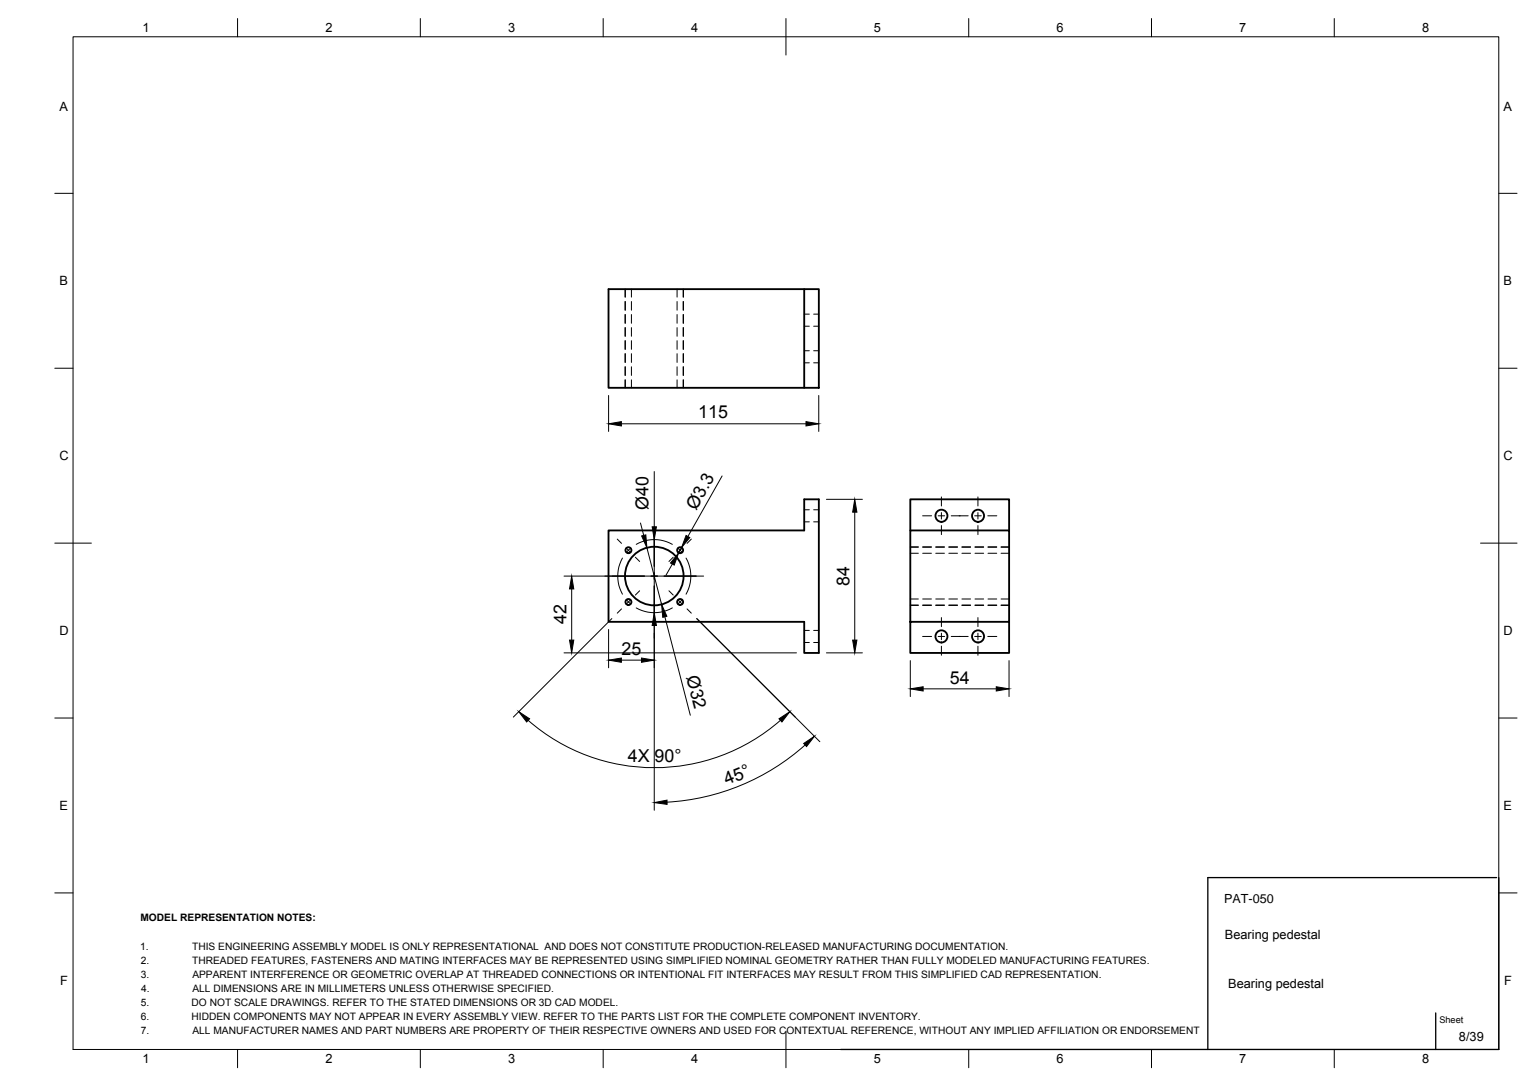
ISO-10303-21;
HEADER;
/* Generated by software containing ST-Developer
 * from STEP Tools, Inc. (www.steptools.com) 
 */

FILE_DESCRIPTION(
/* description */ ('Hand wheel with handle and shaft collar'),
/* implementation_level */ '2;1');

FILE_NAME(
/* name */ 'Bearing pedestal.step',
/* time_stamp */ '2026-10-28T03:23:19-07:00',
/* author */ (''),
/* organization */ (''),
/* preprocessor_version */ 'ST-DEVELOPER v20.2',
/* originating_system */ 'Autodesk Translation Framework v15.17.0.0',
/* authorisation */ '');

FILE_SCHEMA (('AUTOMOTIVE_DESIGN { 1 0 10303 214 3 1 1 }'));
ENDSEC;

DATA;
#10=MECHANICAL_DESIGN_GEOMETRIC_PRESENTATION_REPRESENTATION('',(#398),#10510);
#334=SHAPE_REPRESENTATION_RELATIONSHIP('SRR','None',#10650,#366);
#366=ADVANCED_BREP_SHAPE_REPRESENTATION('',(#445),#10477);
#398=STYLED_ITEM('',(#10908),#445);
#445=MANIFOLD_SOLID_BREP('Body1',#5297);
#494=FACE_BOUND('',#1122,.T.);
#495=FACE_BOUND('',#1123,.T.);
#496=FACE_BOUND('',#1125,.T.);
#497=FACE_BOUND('',#1126,.T.);
#498=FACE_BOUND('',#1130,.T.);
#499=FACE_BOUND('',#1131,.T.);
#500=FACE_BOUND('',#1132,.T.);
#501=FACE_BOUND('',#1133,.T.);
#502=FACE_BOUND('',#1134,.T.);
#503=FACE_BOUND('',#1137,.T.);
#504=FACE_BOUND('',#1138,.T.);
#505=FACE_BOUND('',#1139,.T.);
#506=FACE_BOUND('',#1140,.T.);
#507=FACE_BOUND('',#1141,.T.);
#508=FACE_BOUND('',#1145,.T.);
#509=FACE_BOUND('',#1146,.T.);
#510=FACE_BOUND('',#1147,.T.);
#511=FACE_BOUND('',#1148,.T.);
#616=PLANE('',#5760);
#617=PLANE('',#5761);
#618=PLANE('',#5762);
#619=PLANE('',#5763);
#620=PLANE('',#5764);
#621=PLANE('',#5765);
#622=PLANE('',#5766);
#623=PLANE('',#5767);
#624=PLANE('',#5768);
#625=PLANE('',#5769);
#785=FACE_OUTER_BOUND('',#1112,.T.);
#786=FACE_OUTER_BOUND('',#1113,.T.);
#787=FACE_OUTER_BOUND('',#1114,.T.);
#788=FACE_OUTER_BOUND('',#1115,.T.);
#789=FACE_OUTER_BOUND('',#1116,.T.);
#790=FACE_OUTER_BOUND('',#1117,.T.);
#791=FACE_OUTER_BOUND('',#1118,.T.);
#792=FACE_OUTER_BOUND('',#1119,.T.);
#793=FACE_OUTER_BOUND('',#1120,.T.);
#794=FACE_OUTER_BOUND('',#1121,.T.);
#795=FACE_OUTER_BOUND('',#1124,.T.);
#796=FACE_OUTER_BOUND('',#1127,.T.);
#797=FACE_OUTER_BOUND('',#1128,.T.);
#798=FACE_OUTER_BOUND('',#1129,.T.);
#799=FACE_OUTER_BOUND('',#1135,.T.);
#800=FACE_OUTER_BOUND('',#1136,.T.);
#801=FACE_OUTER_BOUND('',#1142,.T.);
#802=FACE_OUTER_BOUND('',#1143,.T.);
#803=FACE_OUTER_BOUND('',#1144,.T.);
#1112=EDGE_LOOP('',(#3653,#3654,#3655,#3656));
#1113=EDGE_LOOP('',(#3657,#3658,#3659,#3660));
#1114=EDGE_LOOP('',(#3661,#3662,#3663,#3664));
#1115=EDGE_LOOP('',(#3665,#3666,#3667,#3668));
#1116=EDGE_LOOP('',(#3669,#3670,#3671,#3672));
#1117=EDGE_LOOP('',(#3673,#3674,#3675,#3676));
#1118=EDGE_LOOP('',(#3677,#3678,#3679,#3680));
#1119=EDGE_LOOP('',(#3681,#3682,#3683,#3684));
#1120=EDGE_LOOP('',(#3685,#3686,#3687,#3688));
#1121=EDGE_LOOP('',(#3689,#3690,#3691,#3692));
#1122=EDGE_LOOP('',(#3693));
#1123=EDGE_LOOP('',(#3694));
#1124=EDGE_LOOP('',(#3695,#3696,#3697,#3698));
#1125=EDGE_LOOP('',(#3699));
#1126=EDGE_LOOP('',(#3700));
#1127=EDGE_LOOP('',(#3701,#3702,#3703,#3704));
#1128=EDGE_LOOP('',(#3705,#3706,#3707,#3708));
#1129=EDGE_LOOP('',(#3709,#3710,#3711,#3712,#3713,#3714,#3715,#3716));
#1130=EDGE_LOOP('',(#3717));
#1131=EDGE_LOOP('',(#3718));
#1132=EDGE_LOOP('',(#3719));
#1133=EDGE_LOOP('',(#3720));
#1134=EDGE_LOOP('',(#3721));
#1135=EDGE_LOOP('',(#3722,#3723,#3724,#3725));
#1136=EDGE_LOOP('',(#3726,#3727,#3728,#3729,#3730,#3731,#3732,#3733));
#1137=EDGE_LOOP('',(#3734));
#1138=EDGE_LOOP('',(#3735));
#1139=EDGE_LOOP('',(#3736));
#1140=EDGE_LOOP('',(#3737));
#1141=EDGE_LOOP('',(#3738));
#1142=EDGE_LOOP('',(#3739,#3740,#3741,#3742));
#1143=EDGE_LOOP('',(#3743,#3744,#3745,#3746));
#1144=EDGE_LOOP('',(#3747,#3748,#3749,#3750));
#1145=EDGE_LOOP('',(#3751));
#1146=EDGE_LOOP('',(#3752));
#1147=EDGE_LOOP('',(#3753));
#1148=EDGE_LOOP('',(#3754));
#1553=LINE('',#8285,#1863);
#1554=LINE('',#8291,#1864);
#1555=LINE('',#8297,#1865);
#1556=LINE('',#8303,#1866);
#1557=LINE('',#8309,#1867);
#1558=LINE('',#8315,#1868);
#1559=LINE('',#8321,#1869);
#1560=LINE('',#8327,#1870);
#1561=LINE('',#8333,#1871);
#1562=LINE('',#8338,#1872);
#1563=LINE('',#8340,#1873);
#1564=LINE('',#8342,#1874);
#1565=LINE('',#8343,#1875);
#1566=LINE('',#8347,#1876);
#1567=LINE('',#8349,#1877);
#1568=LINE('',#8351,#1878);
#1569=LINE('',#8352,#1879);
#1570=LINE('',#8355,#1880);
#1571=LINE('',#8357,#1881);
#1572=LINE('',#8358,#1882);
#1573=LINE('',#8361,#1883);
#1574=LINE('',#8363,#1884);
#1575=LINE('',#8364,#1885);
#1576=LINE('',#8367,#1886);
#1577=LINE('',#8369,#1887);
#1578=LINE('',#8370,#1888);
#1579=LINE('',#8371,#1889);
#1580=LINE('',#8374,#1890);
#1581=LINE('',#8375,#1891);
#1582=LINE('',#8378,#1892);
#1583=LINE('',#8379,#1893);
#1584=LINE('',#8380,#1894);
#1585=LINE('',#8382,#1895);
#1863=VECTOR('',#6535,0.165);
#1864=VECTOR('',#6542,0.165);
#1865=VECTOR('',#6549,0.165);
#1866=VECTOR('',#6556,0.165);
#1867=VECTOR('',#6563,0.33);
#1868=VECTOR('',#6570,0.33);
#1869=VECTOR('',#6577,0.33);
#1870=VECTOR('',#6584,0.33);
#1871=VECTOR('',#6591,1.6);
#1872=VECTOR('',#6596,1.);
#1873=VECTOR('',#6597,1.);
#1874=VECTOR('',#6598,1.);
#1875=VECTOR('',#6599,1.);
#1876=VECTOR('',#6602,1.);
#1877=VECTOR('',#6603,1.);
#1878=VECTOR('',#6604,1.);
#1879=VECTOR('',#6605,1.);
#1880=VECTOR('',#6608,1.);
#1881=VECTOR('',#6609,1.);
#1882=VECTOR('',#6610,1.);
#1883=VECTOR('',#6613,1.);
#1884=VECTOR('',#6614,1.);
#1885=VECTOR('',#6615,1.);
#1886=VECTOR('',#6618,1.);
#1887=VECTOR('',#6619,1.);
#1888=VECTOR('',#6620,1.);
#1889=VECTOR('',#6621,1.);
#1890=VECTOR('',#6624,1.);
#1891=VECTOR('',#6625,1.);
#1892=VECTOR('',#6628,1.);
#1893=VECTOR('',#6629,1.);
#1894=VECTOR('',#6630,1.);
#1895=VECTOR('',#6633,1.);
#2141=CIRCLE('',#5734,0.165);
#2142=CIRCLE('',#5735,0.165);
#2143=CIRCLE('',#5737,0.165);
#2144=CIRCLE('',#5738,0.165);
#2145=CIRCLE('',#5740,0.165);
#2146=CIRCLE('',#5741,0.165);
#2147=CIRCLE('',#5743,0.165);
#2148=CIRCLE('',#5744,0.165);
#2149=CIRCLE('',#5746,0.33);
#2150=CIRCLE('',#5747,0.33);
#2151=CIRCLE('',#5749,0.33);
#2152=CIRCLE('',#5750,0.33);
#2153=CIRCLE('',#5752,0.33);
#2154=CIRCLE('',#5753,0.33);
#2155=CIRCLE('',#5755,0.33);
#2156=CIRCLE('',#5756,0.33);
#2157=CIRCLE('',#5758,1.6);
#2158=CIRCLE('',#5759,1.6);
#2476=VERTEX_POINT('',#8282);
#2477=VERTEX_POINT('',#8284);
#2478=VERTEX_POINT('',#8288);
#2479=VERTEX_POINT('',#8290);
#2480=VERTEX_POINT('',#8294);
#2481=VERTEX_POINT('',#8296);
#2482=VERTEX_POINT('',#8300);
#2483=VERTEX_POINT('',#8302);
#2484=VERTEX_POINT('',#8306);
#2485=VERTEX_POINT('',#8308);
#2486=VERTEX_POINT('',#8312);
#2487=VERTEX_POINT('',#8314);
#2488=VERTEX_POINT('',#8318);
#2489=VERTEX_POINT('',#8320);
#2490=VERTEX_POINT('',#8324);
#2491=VERTEX_POINT('',#8326);
#2492=VERTEX_POINT('',#8330);
#2493=VERTEX_POINT('',#8332);
#2494=VERTEX_POINT('',#8336);
#2495=VERTEX_POINT('',#8337);
#2496=VERTEX_POINT('',#8339);
#2497=VERTEX_POINT('',#8341);
#2498=VERTEX_POINT('',#8345);
#2499=VERTEX_POINT('',#8346);
#2500=VERTEX_POINT('',#8348);
#2501=VERTEX_POINT('',#8350);
#2502=VERTEX_POINT('',#8354);
#2503=VERTEX_POINT('',#8356);
#2504=VERTEX_POINT('',#8360);
#2505=VERTEX_POINT('',#8362);
#2506=VERTEX_POINT('',#8366);
#2507=VERTEX_POINT('',#8368);
#2508=VERTEX_POINT('',#8373);
#2509=VERTEX_POINT('',#8377);
#2944=EDGE_CURVE('',#2476,#2476,#2141,.T.);
#2945=EDGE_CURVE('',#2476,#2477,#1553,.T.);
#2946=EDGE_CURVE('',#2477,#2477,#2142,.T.);
#2947=EDGE_CURVE('',#2478,#2478,#2143,.T.);
#2948=EDGE_CURVE('',#2478,#2479,#1554,.T.);
#2949=EDGE_CURVE('',#2479,#2479,#2144,.T.);
#2950=EDGE_CURVE('',#2480,#2480,#2145,.T.);
#2951=EDGE_CURVE('',#2480,#2481,#1555,.T.);
#2952=EDGE_CURVE('',#2481,#2481,#2146,.T.);
#2953=EDGE_CURVE('',#2482,#2482,#2147,.T.);
#2954=EDGE_CURVE('',#2482,#2483,#1556,.T.);
#2955=EDGE_CURVE('',#2483,#2483,#2148,.T.);
#2956=EDGE_CURVE('',#2484,#2484,#2149,.T.);
#2957=EDGE_CURVE('',#2484,#2485,#1557,.T.);
#2958=EDGE_CURVE('',#2485,#2485,#2150,.T.);
#2959=EDGE_CURVE('',#2486,#2486,#2151,.T.);
#2960=EDGE_CURVE('',#2486,#2487,#1558,.T.);
#2961=EDGE_CURVE('',#2487,#2487,#2152,.T.);
#2962=EDGE_CURVE('',#2488,#2488,#2153,.T.);
#2963=EDGE_CURVE('',#2488,#2489,#1559,.T.);
#2964=EDGE_CURVE('',#2489,#2489,#2154,.T.);
#2965=EDGE_CURVE('',#2490,#2490,#2155,.T.);
#2966=EDGE_CURVE('',#2490,#2491,#1560,.T.);
#2967=EDGE_CURVE('',#2491,#2491,#2156,.T.);
#2968=EDGE_CURVE('',#2492,#2492,#2157,.T.);
#2969=EDGE_CURVE('',#2492,#2493,#1561,.T.);
#2970=EDGE_CURVE('',#2493,#2493,#2158,.T.);
#2971=EDGE_CURVE('',#2494,#2495,#1562,.T.);
#2972=EDGE_CURVE('',#2496,#2494,#1563,.T.);
#2973=EDGE_CURVE('',#2496,#2497,#1564,.T.);
#2974=EDGE_CURVE('',#2495,#2497,#1565,.T.);
#2975=EDGE_CURVE('',#2498,#2499,#1566,.T.);
#2976=EDGE_CURVE('',#2500,#2498,#1567,.T.);
#2977=EDGE_CURVE('',#2501,#2500,#1568,.T.);
#2978=EDGE_CURVE('',#2499,#2501,#1569,.T.);
#2979=EDGE_CURVE('',#2501,#2502,#1570,.T.);
#2980=EDGE_CURVE('',#2503,#2500,#1571,.T.);
#2981=EDGE_CURVE('',#2502,#2503,#1572,.T.);
#2982=EDGE_CURVE('',#2504,#2496,#1573,.T.);
#2983=EDGE_CURVE('',#2504,#2505,#1574,.T.);
#2984=EDGE_CURVE('',#2497,#2505,#1575,.T.);
#2985=EDGE_CURVE('',#2494,#2506,#1576,.T.);
#2986=EDGE_CURVE('',#2507,#2506,#1577,.T.);
#2987=EDGE_CURVE('',#2499,#2507,#1578,.T.);
#2988=EDGE_CURVE('',#2502,#2504,#1579,.T.);
#2989=EDGE_CURVE('',#2495,#2508,#1580,.T.);
#2990=EDGE_CURVE('',#2506,#2508,#1581,.T.);
#2991=EDGE_CURVE('',#2498,#2509,#1582,.T.);
#2992=EDGE_CURVE('',#2508,#2509,#1583,.T.);
#2993=EDGE_CURVE('',#2505,#2503,#1584,.T.);
#2994=EDGE_CURVE('',#2509,#2507,#1585,.T.);
#3653=ORIENTED_EDGE('',*,*,#2944,.F.);
#3654=ORIENTED_EDGE('',*,*,#2945,.T.);
#3655=ORIENTED_EDGE('',*,*,#2946,.F.);
#3656=ORIENTED_EDGE('',*,*,#2945,.F.);
#3657=ORIENTED_EDGE('',*,*,#2947,.F.);
#3658=ORIENTED_EDGE('',*,*,#2948,.T.);
#3659=ORIENTED_EDGE('',*,*,#2949,.F.);
#3660=ORIENTED_EDGE('',*,*,#2948,.F.);
#3661=ORIENTED_EDGE('',*,*,#2950,.F.);
#3662=ORIENTED_EDGE('',*,*,#2951,.T.);
#3663=ORIENTED_EDGE('',*,*,#2952,.F.);
#3664=ORIENTED_EDGE('',*,*,#2951,.F.);
#3665=ORIENTED_EDGE('',*,*,#2953,.F.);
#3666=ORIENTED_EDGE('',*,*,#2954,.T.);
#3667=ORIENTED_EDGE('',*,*,#2955,.F.);
#3668=ORIENTED_EDGE('',*,*,#2954,.F.);
#3669=ORIENTED_EDGE('',*,*,#2956,.F.);
#3670=ORIENTED_EDGE('',*,*,#2957,.T.);
#3671=ORIENTED_EDGE('',*,*,#2958,.F.);
#3672=ORIENTED_EDGE('',*,*,#2957,.F.);
#3673=ORIENTED_EDGE('',*,*,#2959,.F.);
#3674=ORIENTED_EDGE('',*,*,#2960,.T.);
#3675=ORIENTED_EDGE('',*,*,#2961,.F.);
#3676=ORIENTED_EDGE('',*,*,#2960,.F.);
#3677=ORIENTED_EDGE('',*,*,#2962,.F.);
#3678=ORIENTED_EDGE('',*,*,#2963,.T.);
#3679=ORIENTED_EDGE('',*,*,#2964,.F.);
#3680=ORIENTED_EDGE('',*,*,#2963,.F.);
#3681=ORIENTED_EDGE('',*,*,#2965,.F.);
#3682=ORIENTED_EDGE('',*,*,#2966,.T.);
#3683=ORIENTED_EDGE('',*,*,#2967,.F.);
#3684=ORIENTED_EDGE('',*,*,#2966,.F.);
#3685=ORIENTED_EDGE('',*,*,#2968,.F.);
#3686=ORIENTED_EDGE('',*,*,#2969,.T.);
#3687=ORIENTED_EDGE('',*,*,#2970,.F.);
#3688=ORIENTED_EDGE('',*,*,#2969,.F.);
#3689=ORIENTED_EDGE('',*,*,#2971,.F.);
#3690=ORIENTED_EDGE('',*,*,#2972,.F.);
#3691=ORIENTED_EDGE('',*,*,#2973,.T.);
#3692=ORIENTED_EDGE('',*,*,#2974,.F.);
#3693=ORIENTED_EDGE('',*,*,#2958,.T.);
#3694=ORIENTED_EDGE('',*,*,#2967,.T.);
#3695=ORIENTED_EDGE('',*,*,#2975,.F.);
#3696=ORIENTED_EDGE('',*,*,#2976,.F.);
#3697=ORIENTED_EDGE('',*,*,#2977,.F.);
#3698=ORIENTED_EDGE('',*,*,#2978,.F.);
#3699=ORIENTED_EDGE('',*,*,#2961,.T.);
#3700=ORIENTED_EDGE('',*,*,#2964,.T.);
#3701=ORIENTED_EDGE('',*,*,#2979,.F.);
#3702=ORIENTED_EDGE('',*,*,#2977,.T.);
#3703=ORIENTED_EDGE('',*,*,#2980,.F.);
#3704=ORIENTED_EDGE('',*,*,#2981,.F.);
#3705=ORIENTED_EDGE('',*,*,#2982,.F.);
#3706=ORIENTED_EDGE('',*,*,#2983,.T.);
#3707=ORIENTED_EDGE('',*,*,#2984,.F.);
#3708=ORIENTED_EDGE('',*,*,#2973,.F.);
#3709=ORIENTED_EDGE('',*,*,#2985,.T.);
#3710=ORIENTED_EDGE('',*,*,#2986,.F.);
#3711=ORIENTED_EDGE('',*,*,#2987,.F.);
#3712=ORIENTED_EDGE('',*,*,#2978,.T.);
#3713=ORIENTED_EDGE('',*,*,#2979,.T.);
#3714=ORIENTED_EDGE('',*,*,#2988,.T.);
#3715=ORIENTED_EDGE('',*,*,#2982,.T.);
#3716=ORIENTED_EDGE('',*,*,#2972,.T.);
#3717=ORIENTED_EDGE('',*,*,#2968,.T.);
#3718=ORIENTED_EDGE('',*,*,#2953,.T.);
#3719=ORIENTED_EDGE('',*,*,#2950,.T.);
#3720=ORIENTED_EDGE('',*,*,#2947,.T.);
#3721=ORIENTED_EDGE('',*,*,#2944,.T.);
#3722=ORIENTED_EDGE('',*,*,#2971,.T.);
#3723=ORIENTED_EDGE('',*,*,#2989,.T.);
#3724=ORIENTED_EDGE('',*,*,#2990,.F.);
#3725=ORIENTED_EDGE('',*,*,#2985,.F.);
#3726=ORIENTED_EDGE('',*,*,#2991,.T.);
#3727=ORIENTED_EDGE('',*,*,#2992,.F.);
#3728=ORIENTED_EDGE('',*,*,#2989,.F.);
#3729=ORIENTED_EDGE('',*,*,#2974,.T.);
#3730=ORIENTED_EDGE('',*,*,#2984,.T.);
#3731=ORIENTED_EDGE('',*,*,#2993,.T.);
#3732=ORIENTED_EDGE('',*,*,#2980,.T.);
#3733=ORIENTED_EDGE('',*,*,#2976,.T.);
#3734=ORIENTED_EDGE('',*,*,#2970,.T.);
#3735=ORIENTED_EDGE('',*,*,#2955,.T.);
#3736=ORIENTED_EDGE('',*,*,#2952,.T.);
#3737=ORIENTED_EDGE('',*,*,#2949,.T.);
#3738=ORIENTED_EDGE('',*,*,#2946,.T.);
#3739=ORIENTED_EDGE('',*,*,#2975,.T.);
#3740=ORIENTED_EDGE('',*,*,#2987,.T.);
#3741=ORIENTED_EDGE('',*,*,#2994,.F.);
#3742=ORIENTED_EDGE('',*,*,#2991,.F.);
#3743=ORIENTED_EDGE('',*,*,#2994,.T.);
#3744=ORIENTED_EDGE('',*,*,#2986,.T.);
#3745=ORIENTED_EDGE('',*,*,#2990,.T.);
#3746=ORIENTED_EDGE('',*,*,#2992,.T.);
#3747=ORIENTED_EDGE('',*,*,#2993,.F.);
#3748=ORIENTED_EDGE('',*,*,#2983,.F.);
#3749=ORIENTED_EDGE('',*,*,#2988,.F.);
#3750=ORIENTED_EDGE('',*,*,#2981,.T.);
#3751=ORIENTED_EDGE('',*,*,#2956,.T.);
#3752=ORIENTED_EDGE('',*,*,#2959,.T.);
#3753=ORIENTED_EDGE('',*,*,#2962,.T.);
#3754=ORIENTED_EDGE('',*,*,#2965,.T.);
#4883=CYLINDRICAL_SURFACE('',#5733,0.165);
#4884=CYLINDRICAL_SURFACE('',#5736,0.165);
#4885=CYLINDRICAL_SURFACE('',#5739,0.165);
#4886=CYLINDRICAL_SURFACE('',#5742,0.165);
#4887=CYLINDRICAL_SURFACE('',#5745,0.33);
#4888=CYLINDRICAL_SURFACE('',#5748,0.33);
#4889=CYLINDRICAL_SURFACE('',#5751,0.33);
#4890=CYLINDRICAL_SURFACE('',#5754,0.33);
#4891=CYLINDRICAL_SURFACE('',#5757,1.6);
#4997=ADVANCED_FACE('',(#785),#4883,.F.);
#4998=ADVANCED_FACE('',(#786),#4884,.F.);
#4999=ADVANCED_FACE('',(#787),#4885,.F.);
#5000=ADVANCED_FACE('',(#788),#4886,.F.);
#5001=ADVANCED_FACE('',(#789),#4887,.F.);
#5002=ADVANCED_FACE('',(#790),#4888,.F.);
#5003=ADVANCED_FACE('',(#791),#4889,.F.);
#5004=ADVANCED_FACE('',(#792),#4890,.F.);
#5005=ADVANCED_FACE('',(#793),#4891,.F.);
#5006=ADVANCED_FACE('',(#794,#494,#495),#616,.T.);
#5007=ADVANCED_FACE('',(#795,#496,#497),#617,.T.);
#5008=ADVANCED_FACE('',(#796),#618,.T.);
#5009=ADVANCED_FACE('',(#797),#619,.T.);
#5010=ADVANCED_FACE('',(#798,#498,#499,#500,#501,#502),#620,.T.);
#5011=ADVANCED_FACE('',(#799),#621,.T.);
#5012=ADVANCED_FACE('',(#800,#503,#504,#505,#506,#507),#622,.T.);
#5013=ADVANCED_FACE('',(#801),#623,.T.);
#5014=ADVANCED_FACE('',(#802),#624,.T.);
#5015=ADVANCED_FACE('',(#803,#508,#509,#510,#511),#625,.F.);
#5297=CLOSED_SHELL('',(#4997,#4998,#4999,#5000,#5001,#5002,#5003,#5004,
#5005,#5006,#5007,#5008,#5009,#5010,#5011,#5012,#5013,#5014,#5015));
#5732=AXIS2_PLACEMENT_3D('',#8280,#6529,#6530);
#5733=AXIS2_PLACEMENT_3D('',#8281,#6531,#6532);
#5734=AXIS2_PLACEMENT_3D('',#8283,#6533,#6534);
#5735=AXIS2_PLACEMENT_3D('',#8286,#6536,#6537);
#5736=AXIS2_PLACEMENT_3D('',#8287,#6538,#6539);
#5737=AXIS2_PLACEMENT_3D('',#8289,#6540,#6541);
#5738=AXIS2_PLACEMENT_3D('',#8292,#6543,#6544);
#5739=AXIS2_PLACEMENT_3D('',#8293,#6545,#6546);
#5740=AXIS2_PLACEMENT_3D('',#8295,#6547,#6548);
#5741=AXIS2_PLACEMENT_3D('',#8298,#6550,#6551);
#5742=AXIS2_PLACEMENT_3D('',#8299,#6552,#6553);
#5743=AXIS2_PLACEMENT_3D('',#8301,#6554,#6555);
#5744=AXIS2_PLACEMENT_3D('',#8304,#6557,#6558);
#5745=AXIS2_PLACEMENT_3D('',#8305,#6559,#6560);
#5746=AXIS2_PLACEMENT_3D('',#8307,#6561,#6562);
#5747=AXIS2_PLACEMENT_3D('',#8310,#6564,#6565);
#5748=AXIS2_PLACEMENT_3D('',#8311,#6566,#6567);
#5749=AXIS2_PLACEMENT_3D('',#8313,#6568,#6569);
#5750=AXIS2_PLACEMENT_3D('',#8316,#6571,#6572);
#5751=AXIS2_PLACEMENT_3D('',#8317,#6573,#6574);
#5752=AXIS2_PLACEMENT_3D('',#8319,#6575,#6576);
#5753=AXIS2_PLACEMENT_3D('',#8322,#6578,#6579);
#5754=AXIS2_PLACEMENT_3D('',#8323,#6580,#6581);
#5755=AXIS2_PLACEMENT_3D('',#8325,#6582,#6583);
#5756=AXIS2_PLACEMENT_3D('',#8328,#6585,#6586);
#5757=AXIS2_PLACEMENT_3D('',#8329,#6587,#6588);
#5758=AXIS2_PLACEMENT_3D('',#8331,#6589,#6590);
#5759=AXIS2_PLACEMENT_3D('',#8334,#6592,#6593);
#5760=AXIS2_PLACEMENT_3D('',#8335,#6594,#6595);
#5761=AXIS2_PLACEMENT_3D('',#8344,#6600,#6601);
#5762=AXIS2_PLACEMENT_3D('',#8353,#6606,#6607);
#5763=AXIS2_PLACEMENT_3D('',#8359,#6611,#6612);
#5764=AXIS2_PLACEMENT_3D('',#8365,#6616,#6617);
#5765=AXIS2_PLACEMENT_3D('',#8372,#6622,#6623);
#5766=AXIS2_PLACEMENT_3D('',#8376,#6626,#6627);
#5767=AXIS2_PLACEMENT_3D('',#8381,#6631,#6632);
#5768=AXIS2_PLACEMENT_3D('',#8383,#6634,#6635);
#5769=AXIS2_PLACEMENT_3D('',#8384,#6636,#6637);
#6529=DIRECTION('axis',(0.,0.,1.));
#6530=DIRECTION('refdir',(1.,0.,0.));
#6531=DIRECTION('center_axis',(0.,1.,0.));
#6532=DIRECTION('ref_axis',(1.,0.,0.));
#6533=DIRECTION('center_axis',(0.,1.,0.));
#6534=DIRECTION('ref_axis',(1.,0.,0.));
#6535=DIRECTION('',(0.,1.,0.));
#6536=DIRECTION('center_axis',(0.,-1.,0.));
#6537=DIRECTION('ref_axis',(1.,0.,0.));
#6538=DIRECTION('center_axis',(0.,1.,0.));
#6539=DIRECTION('ref_axis',(1.,0.,0.));
#6540=DIRECTION('center_axis',(0.,1.,0.));
#6541=DIRECTION('ref_axis',(1.,0.,0.));
#6542=DIRECTION('',(0.,1.,0.));
#6543=DIRECTION('center_axis',(0.,-1.,0.));
#6544=DIRECTION('ref_axis',(1.,0.,0.));
#6545=DIRECTION('center_axis',(0.,1.,0.));
#6546=DIRECTION('ref_axis',(1.,0.,0.));
#6547=DIRECTION('center_axis',(0.,1.,0.));
#6548=DIRECTION('ref_axis',(1.,0.,0.));
#6549=DIRECTION('',(0.,1.,0.));
#6550=DIRECTION('center_axis',(0.,-1.,0.));
#6551=DIRECTION('ref_axis',(1.,0.,0.));
#6552=DIRECTION('center_axis',(0.,1.,0.));
#6553=DIRECTION('ref_axis',(1.,0.,0.));
#6554=DIRECTION('center_axis',(0.,1.,0.));
#6555=DIRECTION('ref_axis',(1.,0.,0.));
#6556=DIRECTION('',(0.,1.,0.));
#6557=DIRECTION('center_axis',(0.,-1.,0.));
#6558=DIRECTION('ref_axis',(1.,0.,0.));
#6559=DIRECTION('center_axis',(0.,0.,1.));
#6560=DIRECTION('ref_axis',(1.,0.,0.));
#6561=DIRECTION('center_axis',(0.,0.,1.));
#6562=DIRECTION('ref_axis',(1.,0.,0.));
#6563=DIRECTION('',(0.,0.,1.));
#6564=DIRECTION('center_axis',(0.,0.,-1.));
#6565=DIRECTION('ref_axis',(1.,0.,0.));
#6566=DIRECTION('center_axis',(0.,0.,1.));
#6567=DIRECTION('ref_axis',(1.,0.,0.));
#6568=DIRECTION('center_axis',(0.,0.,1.));
#6569=DIRECTION('ref_axis',(1.,0.,0.));
#6570=DIRECTION('',(0.,0.,1.));
#6571=DIRECTION('center_axis',(0.,0.,-1.));
#6572=DIRECTION('ref_axis',(1.,0.,0.));
#6573=DIRECTION('center_axis',(0.,0.,1.));
#6574=DIRECTION('ref_axis',(1.,0.,0.));
#6575=DIRECTION('center_axis',(0.,0.,1.));
#6576=DIRECTION('ref_axis',(1.,0.,0.));
#6577=DIRECTION('',(0.,0.,1.));
#6578=DIRECTION('center_axis',(0.,0.,-1.));
#6579=DIRECTION('ref_axis',(1.,0.,0.));
#6580=DIRECTION('center_axis',(0.,0.,1.));
#6581=DIRECTION('ref_axis',(1.,0.,0.));
#6582=DIRECTION('center_axis',(0.,0.,1.));
#6583=DIRECTION('ref_axis',(1.,0.,0.));
#6584=DIRECTION('',(0.,0.,1.));
#6585=DIRECTION('center_axis',(0.,0.,-1.));
#6586=DIRECTION('ref_axis',(1.,0.,0.));
#6587=DIRECTION('center_axis',(0.,1.,0.));
#6588=DIRECTION('ref_axis',(1.,0.,0.));
#6589=DIRECTION('center_axis',(0.,1.,0.));
#6590=DIRECTION('ref_axis',(1.,0.,0.));
#6591=DIRECTION('',(0.,1.,0.));
#6592=DIRECTION('center_axis',(0.,-1.,0.));
#6593=DIRECTION('ref_axis',(1.,0.,0.));
#6594=DIRECTION('center_axis',(0.,0.,1.));
#6595=DIRECTION('ref_axis',(1.,0.,0.));
#6596=DIRECTION('',(0.,1.,0.));
#6597=DIRECTION('',(-1.,0.,0.));
#6598=DIRECTION('',(0.,1.,0.));
#6599=DIRECTION('',(1.,0.,0.));
#6600=DIRECTION('center_axis',(0.,0.,1.));
#6601=DIRECTION('ref_axis',(1.,0.,0.));
#6602=DIRECTION('',(0.,-1.,0.));
#6603=DIRECTION('',(1.,0.,0.));
#6604=DIRECTION('',(0.,1.,0.));
#6605=DIRECTION('',(-1.,0.,0.));
#6606=DIRECTION('center_axis',(-1.,0.,0.));
#6607=DIRECTION('ref_axis',(0.,0.,1.));
#6608=DIRECTION('',(0.,0.,-1.));
#6609=DIRECTION('',(0.,0.,1.));
#6610=DIRECTION('',(0.,1.,0.));
#6611=DIRECTION('center_axis',(1.,0.,0.));
#6612=DIRECTION('ref_axis',(0.,0.,-1.));
#6613=DIRECTION('',(0.,0.,1.));
#6614=DIRECTION('',(0.,1.,0.));
#6615=DIRECTION('',(0.,0.,-1.));
#6616=DIRECTION('center_axis',(0.,-1.,0.));
#6617=DIRECTION('ref_axis',(1.,0.,0.));
#6618=DIRECTION('',(0.,0.,1.));
#6619=DIRECTION('',(1.,0.,0.));
#6620=DIRECTION('',(0.,0.,1.));
#6621=DIRECTION('',(1.,0.,0.));
#6622=DIRECTION('center_axis',(1.,0.,0.));
#6623=DIRECTION('ref_axis',(0.,1.,0.));
#6624=DIRECTION('',(0.,0.,1.));
#6625=DIRECTION('',(0.,1.,0.));
#6626=DIRECTION('center_axis',(0.,1.,0.));
#6627=DIRECTION('ref_axis',(-1.,0.,0.));
#6628=DIRECTION('',(0.,0.,1.));
#6629=DIRECTION('',(-1.,0.,0.));
#6630=DIRECTION('',(-1.,0.,0.));
#6631=DIRECTION('center_axis',(-1.,0.,0.));
#6632=DIRECTION('ref_axis',(0.,-1.,0.));
#6633=DIRECTION('',(0.,-1.,0.));
#6634=DIRECTION('center_axis',(0.,0.,1.));
#6635=DIRECTION('ref_axis',(1.,0.,0.));
#6636=DIRECTION('center_axis',(0.,0.,1.));
#6637=DIRECTION('ref_axis',(1.,0.,0.));
#8280=CARTESIAN_POINT('',(0.,0.,0.));
#8281=CARTESIAN_POINT('Origin',(-1.4142135623731,-0.8,8.5857864376269));
#8282=CARTESIAN_POINT('',(-1.5792135623731,-0.7,8.5857864376269));
#8283=CARTESIAN_POINT('Origin',(-1.4142135623731,-0.7,8.5857864376269));
#8284=CARTESIAN_POINT('',(-1.5792135623731,4.7,8.5857864376269));
#8285=CARTESIAN_POINT('',(-1.5792135623731,-0.8,8.5857864376269));
#8286=CARTESIAN_POINT('Origin',(-1.4142135623731,4.7,8.5857864376269));
#8287=CARTESIAN_POINT('Origin',(-1.41421356237309,-0.8,11.4142135623731));
#8288=CARTESIAN_POINT('',(-1.57921356237309,-0.7,11.4142135623731));
#8289=CARTESIAN_POINT('Origin',(-1.41421356237309,-0.7,11.4142135623731));
#8290=CARTESIAN_POINT('',(-1.57921356237309,4.7,11.4142135623731));
#8291=CARTESIAN_POINT('',(-1.57921356237309,-0.8,11.4142135623731));
#8292=CARTESIAN_POINT('Origin',(-1.41421356237309,4.7,11.4142135623731));
#8293=CARTESIAN_POINT('Origin',(1.4142135623731,-0.8,11.4142135623731));
#8294=CARTESIAN_POINT('',(1.2492135623731,-0.7,11.4142135623731));
#8295=CARTESIAN_POINT('Origin',(1.4142135623731,-0.7,11.4142135623731));
#8296=CARTESIAN_POINT('',(1.2492135623731,4.7,11.4142135623731));
#8297=CARTESIAN_POINT('',(1.2492135623731,-0.8,11.4142135623731));
#8298=CARTESIAN_POINT('Origin',(1.4142135623731,4.7,11.4142135623731));
#8299=CARTESIAN_POINT('Origin',(1.41421356237309,-0.8,8.5857864376269));
#8300=CARTESIAN_POINT('',(1.24921356237309,-0.7,8.5857864376269));
#8301=CARTESIAN_POINT('Origin',(1.41421356237309,-0.7,8.5857864376269));
#8302=CARTESIAN_POINT('',(1.24921356237309,4.7,8.5857864376269));
#8303=CARTESIAN_POINT('',(1.24921356237309,-0.8,8.5857864376269));
#8304=CARTESIAN_POINT('Origin',(1.41421356237309,4.7,8.5857864376269));
#8305=CARTESIAN_POINT('Origin',(3.3,1.,0.9));
#8306=CARTESIAN_POINT('',(2.97,1.,1.));
#8307=CARTESIAN_POINT('Origin',(3.3,1.,1.));
#8308=CARTESIAN_POINT('',(2.97,1.,1.8));
#8309=CARTESIAN_POINT('',(2.97,1.,0.9));
#8310=CARTESIAN_POINT('Origin',(3.3,1.,1.8));
#8311=CARTESIAN_POINT('Origin',(-3.3,3.,0.9));
#8312=CARTESIAN_POINT('',(-3.63,3.,1.));
#8313=CARTESIAN_POINT('Origin',(-3.3,3.,1.));
#8314=CARTESIAN_POINT('',(-3.63,3.,1.8));
#8315=CARTESIAN_POINT('',(-3.63,3.,0.9));
#8316=CARTESIAN_POINT('Origin',(-3.3,3.,1.8));
#8317=CARTESIAN_POINT('Origin',(-3.3,1.,0.9));
#8318=CARTESIAN_POINT('',(-3.63,1.,1.));
#8319=CARTESIAN_POINT('Origin',(-3.3,1.,1.));
#8320=CARTESIAN_POINT('',(-3.63,1.,1.8));
#8321=CARTESIAN_POINT('',(-3.63,1.,0.9));
#8322=CARTESIAN_POINT('Origin',(-3.3,1.,1.8));
#8323=CARTESIAN_POINT('Origin',(3.3,3.,0.9));
#8324=CARTESIAN_POINT('',(2.97,3.,1.));
#8325=CARTESIAN_POINT('Origin',(3.3,3.,1.));
#8326=CARTESIAN_POINT('',(2.97,3.,1.8));
#8327=CARTESIAN_POINT('',(2.97,3.,0.9));
#8328=CARTESIAN_POINT('Origin',(3.3,3.,1.8));
#8329=CARTESIAN_POINT('Origin',(0.,-0.8,10.));
#8330=CARTESIAN_POINT('',(-1.6,-0.7,10.));
#8331=CARTESIAN_POINT('Origin',(0.,-0.7,10.));
#8332=CARTESIAN_POINT('',(-1.6,4.7,10.));
#8333=CARTESIAN_POINT('',(-1.6,-0.8,10.));
#8334=CARTESIAN_POINT('Origin',(0.,4.7,10.));
#8335=CARTESIAN_POINT('Origin',(-4.2,-0.7,1.8));
#8336=CARTESIAN_POINT('',(2.5,-0.7,1.8));
#8337=CARTESIAN_POINT('',(2.5,4.7,1.8));
#8338=CARTESIAN_POINT('',(2.5,-0.7,1.8));
#8339=CARTESIAN_POINT('',(4.2,-0.7,1.8));
#8340=CARTESIAN_POINT('',(4.2,-0.7,1.8));
#8341=CARTESIAN_POINT('',(4.2,4.7,1.8));
#8342=CARTESIAN_POINT('',(4.2,-0.7,1.8));
#8343=CARTESIAN_POINT('',(4.2,4.7,1.8));
#8344=CARTESIAN_POINT('Origin',(-4.2,-0.7,1.8));
#8345=CARTESIAN_POINT('',(-2.5,4.7,1.8));
#8346=CARTESIAN_POINT('',(-2.5,-0.7,1.8));
#8347=CARTESIAN_POINT('',(-2.5,2.,1.8));
#8348=CARTESIAN_POINT('',(-4.2,4.7,1.8));
#8349=CARTESIAN_POINT('',(4.2,4.7,1.8));
#8350=CARTESIAN_POINT('',(-4.2,-0.7,1.8));
#8351=CARTESIAN_POINT('',(-4.2,-0.7,1.8));
#8352=CARTESIAN_POINT('',(4.2,-0.7,1.8));
#8353=CARTESIAN_POINT('Origin',(-4.2,-0.7,1.));
#8354=CARTESIAN_POINT('',(-4.2,-0.7,1.));
#8355=CARTESIAN_POINT('',(-4.2,-0.7,1.8));
#8356=CARTESIAN_POINT('',(-4.2,4.7,1.));
#8357=CARTESIAN_POINT('',(-4.2,4.7,1.8));
#8358=CARTESIAN_POINT('',(-4.2,-0.7,1.));
#8359=CARTESIAN_POINT('Origin',(4.2,-0.7,1.8));
#8360=CARTESIAN_POINT('',(4.2,-0.7,1.));
#8361=CARTESIAN_POINT('',(4.2,-0.7,1.));
#8362=CARTESIAN_POINT('',(4.2,4.7,1.));
#8363=CARTESIAN_POINT('',(4.2,-0.7,1.));
#8364=CARTESIAN_POINT('',(4.2,4.7,1.));
#8365=CARTESIAN_POINT('Origin',(-2.5,-0.7,1.));
#8366=CARTESIAN_POINT('',(2.5,-0.7,12.5));
#8367=CARTESIAN_POINT('',(2.5,-0.7,1.));
#8368=CARTESIAN_POINT('',(-2.5,-0.7,12.5));
#8369=CARTESIAN_POINT('',(-2.5,-0.7,12.5));
#8370=CARTESIAN_POINT('',(-2.5,-0.7,1.));
#8371=CARTESIAN_POINT('',(-4.2,-0.7,1.));
#8372=CARTESIAN_POINT('Origin',(2.5,-0.7,1.));
#8373=CARTESIAN_POINT('',(2.5,4.7,12.5));
#8374=CARTESIAN_POINT('',(2.5,4.7,1.));
#8375=CARTESIAN_POINT('',(2.5,-0.7,12.5));
#8376=CARTESIAN_POINT('Origin',(2.5,4.7,1.));
#8377=CARTESIAN_POINT('',(-2.5,4.7,12.5));
#8378=CARTESIAN_POINT('',(-2.5,4.7,1.));
#8379=CARTESIAN_POINT('',(2.5,4.7,12.5));
#8380=CARTESIAN_POINT('',(-4.2,4.7,1.));
#8381=CARTESIAN_POINT('Origin',(-2.5,4.7,1.));
#8382=CARTESIAN_POINT('',(-2.5,4.7,12.5));
#8383=CARTESIAN_POINT('Origin',(0.,2.,12.5));
#8384=CARTESIAN_POINT('Origin',(0.,2.,1.));
#10438=UNCERTAINTY_MEASURE_WITH_UNIT(LENGTH_MEASURE(0.001),#10511,
'DISTANCE_ACCURACY_VALUE',
'Maximum model space distance between geometric entities at asserted c
onnectivities');
#10471=UNCERTAINTY_MEASURE_WITH_UNIT(LENGTH_MEASURE(0.001),#10511,
'DISTANCE_ACCURACY_VALUE',
'Maximum model space distance between geometric entities at asserted c
onnectivities');
#10477=(
GEOMETRIC_REPRESENTATION_CONTEXT(3)
GLOBAL_UNCERTAINTY_ASSIGNED_CONTEXT((#10438))
GLOBAL_UNIT_ASSIGNED_CONTEXT((#10511,#10513,#10514))
REPRESENTATION_CONTEXT('','3D')
);
#10510=(
GEOMETRIC_REPRESENTATION_CONTEXT(3)
GLOBAL_UNCERTAINTY_ASSIGNED_CONTEXT((#10471))
GLOBAL_UNIT_ASSIGNED_CONTEXT((#10511,#10513,#10514))
REPRESENTATION_CONTEXT('','3D')
);
#10511=(
LENGTH_UNIT()
NAMED_UNIT(*)
SI_UNIT(.CENTI.,.METRE.)
);
#10513=(
NAMED_UNIT(*)
PLANE_ANGLE_UNIT()
SI_UNIT($,.RADIAN.)
);
#10514=(
NAMED_UNIT(*)
SI_UNIT($,.STERADIAN.)
SOLID_ANGLE_UNIT()
);
#10520=SHAPE_DEFINITION_REPRESENTATION(#10558,#10650);
#10558=PRODUCT_DEFINITION_SHAPE('',$,#10689);
#10650=SHAPE_REPRESENTATION('',(#5732),#10477);
#10683=PRODUCT_DEFINITION_CONTEXT('part definition',#10799,'design');
#10689=PRODUCT_DEFINITION('Bearing pedestal','Bearing pedestal',#10727,
#10683);
#10727=PRODUCT_DEFINITION_FORMATION('',$,#10806);
#10799=APPLICATION_CONTEXT(
'Core Data for Automotive Mechanical Design Process');
#10800=PRODUCT_CONTEXT('part definition',#10799,'mechanical');
#10806=PRODUCT('Bearing pedestal','Bearing pedestal','Bearing pedestal',
(#10800));
#10902=COLOUR_RGB('Grey',0.48,0.52,0.57);
#10903=FILL_AREA_STYLE_COLOUR('',#10902);
#10904=FILL_AREA_STYLE('',(#10903));
#10905=SURFACE_STYLE_FILL_AREA(#10904);
#10906=SURFACE_SIDE_STYLE('',(#10905));
#10907=SURFACE_STYLE_USAGE(.BOTH.,#10906);
#10908=PRESENTATION_STYLE_ASSIGNMENT((#10907));
ENDSEC;
END-ISO-10303-21;
